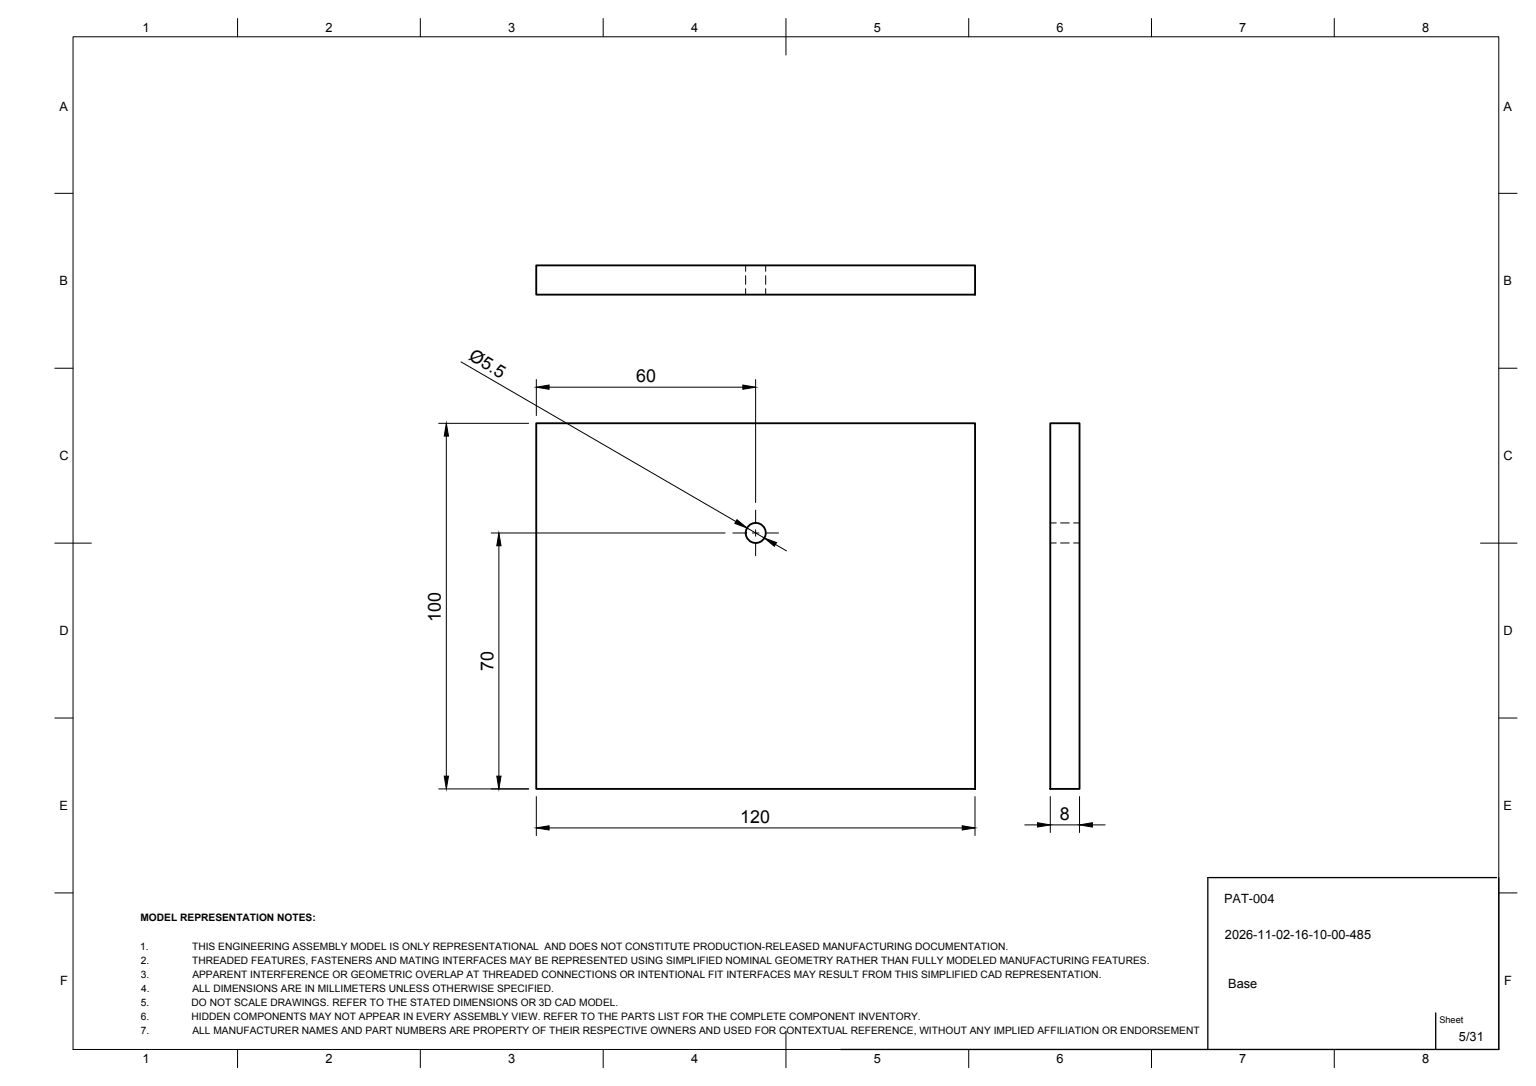
ISO-10303-21;
HEADER;
/* Generated by software containing ST-Developer
 * from STEP Tools, Inc. (www.steptools.com) 
 */

FILE_DESCRIPTION(
/* description */ ('Air blow-off nozzle station'),
/* implementation_level */ '2;1');

FILE_NAME(
/* name */ 'Base.step',
/* time_stamp */ '2026-10-27T10:53:54-07:00',
/* author */ (''),
/* organization */ (''),
/* preprocessor_version */ 'ST-DEVELOPER v20.2',
/* originating_system */ 'Autodesk Translation Framework v15.17.0.0',
/* authorisation */ '');

FILE_SCHEMA (('AUTOMOTIVE_DESIGN { 1 0 10303 214 3 1 1 }'));
ENDSEC;

DATA;
#10=MECHANICAL_DESIGN_GEOMETRIC_PRESENTATION_REPRESENTATION('',(#237),#7897);
#187=SHAPE_REPRESENTATION_RELATIONSHIP('SRR','None',#8001,#212);
#212=ADVANCED_BREP_SHAPE_REPRESENTATION('',(#262),#7868);
#237=STYLED_ITEM('',(#8199),#262);
#262=MANIFOLD_SOLID_BREP('Body1',#4286);
#285=FACE_BOUND('',#802,.T.);
#286=FACE_BOUND('',#804,.T.);
#371=PLANE('',#4595);
#372=PLANE('',#4596);
#373=PLANE('',#4597);
#374=PLANE('',#4598);
#375=PLANE('',#4599);
#376=PLANE('',#4600);
#540=FACE_OUTER_BOUND('',#796,.T.);
#541=FACE_OUTER_BOUND('',#797,.T.);
#542=FACE_OUTER_BOUND('',#798,.T.);
#543=FACE_OUTER_BOUND('',#799,.T.);
#544=FACE_OUTER_BOUND('',#800,.T.);
#545=FACE_OUTER_BOUND('',#801,.T.);
#546=FACE_OUTER_BOUND('',#803,.T.);
#796=EDGE_LOOP('',(#2897,#2898,#2899,#2900));
#797=EDGE_LOOP('',(#2901,#2902,#2903,#2904));
#798=EDGE_LOOP('',(#2905,#2906,#2907,#2908));
#799=EDGE_LOOP('',(#2909,#2910,#2911,#2912));
#800=EDGE_LOOP('',(#2913,#2914,#2915,#2916));
#801=EDGE_LOOP('',(#2917,#2918,#2919,#2920));
#802=EDGE_LOOP('',(#2921));
#803=EDGE_LOOP('',(#2922,#2923,#2924,#2925));
#804=EDGE_LOOP('',(#2926));
#1138=LINE('',#6399,#1492);
#1139=LINE('',#6404,#1493);
#1140=LINE('',#6406,#1494);
#1141=LINE('',#6408,#1495);
#1142=LINE('',#6409,#1496);
#1143=LINE('',#6412,#1497);
#1144=LINE('',#6414,#1498);
#1145=LINE('',#6415,#1499);
#1146=LINE('',#6418,#1500);
#1147=LINE('',#6420,#1501);
#1148=LINE('',#6421,#1502);
#1149=LINE('',#6423,#1503);
#1150=LINE('',#6424,#1504);
#1492=VECTOR('',#5082,0.275);
#1493=VECTOR('',#5087,1.);
#1494=VECTOR('',#5088,1.);
#1495=VECTOR('',#5089,1.);
#1496=VECTOR('',#5090,1.);
#1497=VECTOR('',#5093,1.);
#1498=VECTOR('',#5094,1.);
#1499=VECTOR('',#5095,1.);
#1500=VECTOR('',#5098,1.);
#1501=VECTOR('',#5099,1.);
#1502=VECTOR('',#5100,1.);
#1503=VECTOR('',#5103,1.);
#1504=VECTOR('',#5104,1.);
#1846=CIRCLE('',#4593,0.275);
#1847=CIRCLE('',#4594,0.275);
#2007=VERTEX_POINT('',#6396);
#2008=VERTEX_POINT('',#6398);
#2009=VERTEX_POINT('',#6402);
#2010=VERTEX_POINT('',#6403);
#2011=VERTEX_POINT('',#6405);
#2012=VERTEX_POINT('',#6407);
#2013=VERTEX_POINT('',#6411);
#2014=VERTEX_POINT('',#6413);
#2015=VERTEX_POINT('',#6417);
#2016=VERTEX_POINT('',#6419);
#2366=EDGE_CURVE('',#2007,#2007,#1846,.T.);
#2367=EDGE_CURVE('',#2007,#2008,#1138,.T.);
#2368=EDGE_CURVE('',#2008,#2008,#1847,.T.);
#2369=EDGE_CURVE('',#2009,#2010,#1139,.T.);
#2370=EDGE_CURVE('',#2010,#2011,#1140,.T.);
#2371=EDGE_CURVE('',#2012,#2011,#1141,.T.);
#2372=EDGE_CURVE('',#2009,#2012,#1142,.T.);
#2373=EDGE_CURVE('',#2013,#2009,#1143,.T.);
#2374=EDGE_CURVE('',#2014,#2012,#1144,.T.);
#2375=EDGE_CURVE('',#2013,#2014,#1145,.T.);
#2376=EDGE_CURVE('',#2015,#2013,#1146,.T.);
#2377=EDGE_CURVE('',#2016,#2014,#1147,.T.);
#2378=EDGE_CURVE('',#2015,#2016,#1148,.T.);
#2379=EDGE_CURVE('',#2010,#2015,#1149,.T.);
#2380=EDGE_CURVE('',#2011,#2016,#1150,.T.);
#2897=ORIENTED_EDGE('',*,*,#2366,.F.);
#2898=ORIENTED_EDGE('',*,*,#2367,.T.);
#2899=ORIENTED_EDGE('',*,*,#2368,.F.);
#2900=ORIENTED_EDGE('',*,*,#2367,.F.);
#2901=ORIENTED_EDGE('',*,*,#2369,.T.);
#2902=ORIENTED_EDGE('',*,*,#2370,.T.);
#2903=ORIENTED_EDGE('',*,*,#2371,.F.);
#2904=ORIENTED_EDGE('',*,*,#2372,.F.);
#2905=ORIENTED_EDGE('',*,*,#2373,.T.);
#2906=ORIENTED_EDGE('',*,*,#2372,.T.);
#2907=ORIENTED_EDGE('',*,*,#2374,.F.);
#2908=ORIENTED_EDGE('',*,*,#2375,.F.);
#2909=ORIENTED_EDGE('',*,*,#2376,.T.);
#2910=ORIENTED_EDGE('',*,*,#2375,.T.);
#2911=ORIENTED_EDGE('',*,*,#2377,.F.);
#2912=ORIENTED_EDGE('',*,*,#2378,.F.);
#2913=ORIENTED_EDGE('',*,*,#2379,.T.);
#2914=ORIENTED_EDGE('',*,*,#2378,.T.);
#2915=ORIENTED_EDGE('',*,*,#2380,.F.);
#2916=ORIENTED_EDGE('',*,*,#2370,.F.);
#2917=ORIENTED_EDGE('',*,*,#2380,.T.);
#2918=ORIENTED_EDGE('',*,*,#2377,.T.);
#2919=ORIENTED_EDGE('',*,*,#2374,.T.);
#2920=ORIENTED_EDGE('',*,*,#2371,.T.);
#2921=ORIENTED_EDGE('',*,*,#2368,.T.);
#2922=ORIENTED_EDGE('',*,*,#2379,.F.);
#2923=ORIENTED_EDGE('',*,*,#2369,.F.);
#2924=ORIENTED_EDGE('',*,*,#2373,.F.);
#2925=ORIENTED_EDGE('',*,*,#2376,.F.);
#2926=ORIENTED_EDGE('',*,*,#2366,.T.);
#3959=CYLINDRICAL_SURFACE('',#4592,0.275);
#4030=ADVANCED_FACE('',(#540),#3959,.F.);
#4031=ADVANCED_FACE('',(#541),#371,.T.);
#4032=ADVANCED_FACE('',(#542),#372,.T.);
#4033=ADVANCED_FACE('',(#543),#373,.T.);
#4034=ADVANCED_FACE('',(#544),#374,.T.);
#4035=ADVANCED_FACE('',(#545,#285),#375,.T.);
#4036=ADVANCED_FACE('',(#546,#286),#376,.F.);
#4286=CLOSED_SHELL('',(#4030,#4031,#4032,#4033,#4034,#4035,#4036));
#4591=AXIS2_PLACEMENT_3D('',#6394,#5076,#5077);
#4592=AXIS2_PLACEMENT_3D('',#6395,#5078,#5079);
#4593=AXIS2_PLACEMENT_3D('',#6397,#5080,#5081);
#4594=AXIS2_PLACEMENT_3D('',#6400,#5083,#5084);
#4595=AXIS2_PLACEMENT_3D('',#6401,#5085,#5086);
#4596=AXIS2_PLACEMENT_3D('',#6410,#5091,#5092);
#4597=AXIS2_PLACEMENT_3D('',#6416,#5096,#5097);
#4598=AXIS2_PLACEMENT_3D('',#6422,#5101,#5102);
#4599=AXIS2_PLACEMENT_3D('',#6425,#5105,#5106);
#4600=AXIS2_PLACEMENT_3D('',#6426,#5107,#5108);
#5076=DIRECTION('axis',(0.,0.,1.));
#5077=DIRECTION('refdir',(1.,0.,0.));
#5078=DIRECTION('center_axis',(0.,0.,1.));
#5079=DIRECTION('ref_axis',(1.,0.,0.));
#5080=DIRECTION('center_axis',(0.,0.,1.));
#5081=DIRECTION('ref_axis',(1.,0.,0.));
#5082=DIRECTION('',(0.,0.,1.));
#5083=DIRECTION('center_axis',(0.,0.,-1.));
#5084=DIRECTION('ref_axis',(1.,0.,0.));
#5085=DIRECTION('center_axis',(0.,1.,0.));
#5086=DIRECTION('ref_axis',(-1.,0.,0.));
#5087=DIRECTION('',(-1.,0.,0.));
#5088=DIRECTION('',(0.,0.,1.));
#5089=DIRECTION('',(-1.,0.,0.));
#5090=DIRECTION('',(0.,0.,1.));
#5091=DIRECTION('center_axis',(1.,0.,0.));
#5092=DIRECTION('ref_axis',(0.,1.,0.));
#5093=DIRECTION('',(0.,1.,0.));
#5094=DIRECTION('',(0.,1.,0.));
#5095=DIRECTION('',(0.,0.,1.));
#5096=DIRECTION('center_axis',(0.,-1.,0.));
#5097=DIRECTION('ref_axis',(1.,0.,0.));
#5098=DIRECTION('',(1.,0.,0.));
#5099=DIRECTION('',(1.,0.,0.));
#5100=DIRECTION('',(0.,0.,1.));
#5101=DIRECTION('center_axis',(-1.,0.,0.));
#5102=DIRECTION('ref_axis',(0.,-1.,0.));
#5103=DIRECTION('',(0.,-1.,0.));
#5104=DIRECTION('',(0.,-1.,0.));
#5105=DIRECTION('center_axis',(0.,0.,1.));
#5106=DIRECTION('ref_axis',(1.,0.,0.));
#5107=DIRECTION('center_axis',(0.,0.,1.));
#5108=DIRECTION('ref_axis',(1.,0.,0.));
#6394=CARTESIAN_POINT('',(0.,0.,0.));
#6395=CARTESIAN_POINT('Origin',(0.,3.,-0.1));
#6396=CARTESIAN_POINT('',(-0.275,3.,0.));
#6397=CARTESIAN_POINT('Origin',(0.,3.,0.));
#6398=CARTESIAN_POINT('',(-0.275,3.,0.8));
#6399=CARTESIAN_POINT('',(-0.275,3.,-0.1));
#6400=CARTESIAN_POINT('Origin',(0.,3.,0.8));
#6401=CARTESIAN_POINT('Origin',(6.,6.,0.));
#6402=CARTESIAN_POINT('',(6.,6.,0.));
#6403=CARTESIAN_POINT('',(-6.,6.,0.));
#6404=CARTESIAN_POINT('',(6.,6.,0.));
#6405=CARTESIAN_POINT('',(-6.,6.,0.8));
#6406=CARTESIAN_POINT('',(-6.,6.,0.));
#6407=CARTESIAN_POINT('',(6.,6.,0.8));
#6408=CARTESIAN_POINT('',(6.,6.,0.8));
#6409=CARTESIAN_POINT('',(6.,6.,0.));
#6410=CARTESIAN_POINT('Origin',(6.,-4.,0.));
#6411=CARTESIAN_POINT('',(6.,-4.,0.));
#6412=CARTESIAN_POINT('',(6.,-4.,0.));
#6413=CARTESIAN_POINT('',(6.,-4.,0.8));
#6414=CARTESIAN_POINT('',(6.,-4.,0.8));
#6415=CARTESIAN_POINT('',(6.,-4.,0.));
#6416=CARTESIAN_POINT('Origin',(-6.,-4.,0.));
#6417=CARTESIAN_POINT('',(-6.,-4.,0.));
#6418=CARTESIAN_POINT('',(-6.,-4.,0.));
#6419=CARTESIAN_POINT('',(-6.,-4.,0.8));
#6420=CARTESIAN_POINT('',(-6.,-4.,0.8));
#6421=CARTESIAN_POINT('',(-6.,-4.,0.));
#6422=CARTESIAN_POINT('Origin',(-6.,6.,0.));
#6423=CARTESIAN_POINT('',(-6.,6.,0.));
#6424=CARTESIAN_POINT('',(-6.,6.,0.8));
#6425=CARTESIAN_POINT('Origin',(0.,1.,0.8));
#6426=CARTESIAN_POINT('Origin',(0.,1.,0.));
#7836=UNCERTAINTY_MEASURE_WITH_UNIT(LENGTH_MEASURE(0.001),#7898,
'DISTANCE_ACCURACY_VALUE',
'Maximum model space distance between geometric entities at asserted c
onnectivities');
#7865=UNCERTAINTY_MEASURE_WITH_UNIT(LENGTH_MEASURE(0.001),#7898,
'DISTANCE_ACCURACY_VALUE',
'Maximum model space distance between geometric entities at asserted c
onnectivities');
#7868=(
GEOMETRIC_REPRESENTATION_CONTEXT(3)
GLOBAL_UNCERTAINTY_ASSIGNED_CONTEXT((#7836))
GLOBAL_UNIT_ASSIGNED_CONTEXT((#7898,#7900,#7901))
REPRESENTATION_CONTEXT('','3D')
);
#7897=(
GEOMETRIC_REPRESENTATION_CONTEXT(3)
GLOBAL_UNCERTAINTY_ASSIGNED_CONTEXT((#7865))
GLOBAL_UNIT_ASSIGNED_CONTEXT((#7898,#7900,#7901))
REPRESENTATION_CONTEXT('','3D')
);
#7898=(
LENGTH_UNIT()
NAMED_UNIT(*)
SI_UNIT(.CENTI.,.METRE.)
);
#7900=(
NAMED_UNIT(*)
PLANE_ANGLE_UNIT()
SI_UNIT($,.RADIAN.)
);
#7901=(
NAMED_UNIT(*)
SI_UNIT($,.STERADIAN.)
SOLID_ANGLE_UNIT()
);
#7904=SHAPE_DEFINITION_REPRESENTATION(#7935,#8001);
#7935=PRODUCT_DEFINITION_SHAPE('',$,#8033);
#8001=SHAPE_REPRESENTATION('',(#4591),#7868);
#8030=PRODUCT_DEFINITION_CONTEXT('part definition',#8125,'design');
#8033=PRODUCT_DEFINITION('Base','Base',#8064,#8030);
#8064=PRODUCT_DEFINITION_FORMATION('',$,#8129);
#8125=APPLICATION_CONTEXT(
'Core Data for Automotive Mechanical Design Process');
#8126=PRODUCT_CONTEXT('part definition',#8125,'mechanical');
#8129=PRODUCT('Base','Base','Base',(#8126));
#8193=COLOUR_RGB('Dark Blue',0.08,0.2,0.34);
#8194=FILL_AREA_STYLE_COLOUR('',#8193);
#8195=FILL_AREA_STYLE('',(#8194));
#8196=SURFACE_STYLE_FILL_AREA(#8195);
#8197=SURFACE_SIDE_STYLE('',(#8196));
#8198=SURFACE_STYLE_USAGE(.BOTH.,#8197);
#8199=PRESENTATION_STYLE_ASSIGNMENT((#8198));
ENDSEC;
END-ISO-10303-21;
